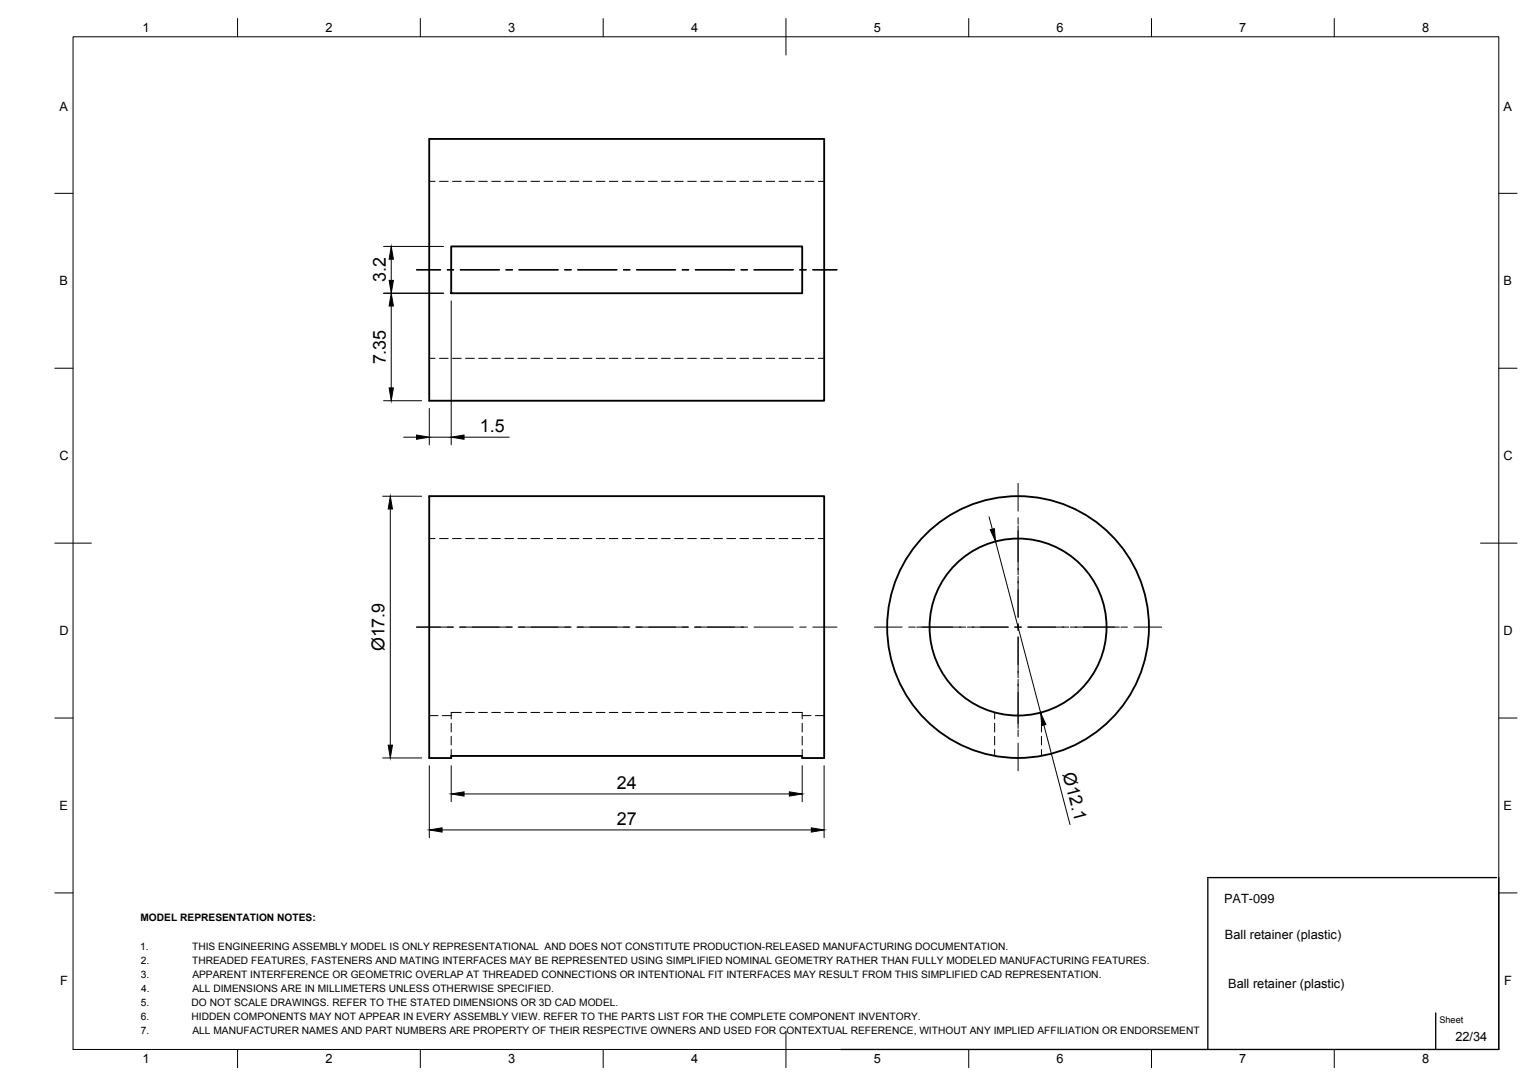
ISO-10303-21;
HEADER;
/* Generated by software containing ST-Developer
 * from STEP Tools, Inc. (www.steptools.com) 
 */

FILE_DESCRIPTION(
/* description */ ('PAT-099'),
/* implementation_level */ '2;1');

FILE_NAME(
/* name */ 'Ball retainer (plastic).step',
/* time_stamp */ '2026-10-29T17:25:42-07:00',
/* author */ (''),
/* organization */ (''),
/* preprocessor_version */ 'ST-DEVELOPER v20.2',
/* originating_system */ 'Autodesk Translation Framework v15.17.0.0',
/* authorisation */ '');

FILE_SCHEMA (('AUTOMOTIVE_DESIGN { 1 0 10303 214 3 1 1 }'));
ENDSEC;

DATA;
#10=MECHANICAL_DESIGN_GEOMETRIC_PRESENTATION_REPRESENTATION('',(#345),#11035);
#295=SHAPE_REPRESENTATION_RELATIONSHIP('SRR','None',#11164,#320);
#320=ADVANCED_BREP_SHAPE_REPRESENTATION('',(#378),#11014);
#345=STYLED_ITEM('',(#11379),#378);
#378=MANIFOLD_SOLID_BREP('Body1',#4713);
#485=FACE_BOUND('',#1151,.T.);
#486=FACE_BOUND('',#1153,.T.);
#487=FACE_BOUND('',#1155,.T.);
#488=FACE_BOUND('',#1157,.T.);
#573=PLANE('',#5293);
#574=PLANE('',#5296);
#575=PLANE('',#5297);
#576=PLANE('',#5300);
#577=PLANE('',#5301);
#578=PLANE('',#5306);
#781=FACE_OUTER_BOUND('',#1146,.T.);
#782=FACE_OUTER_BOUND('',#1147,.T.);
#783=FACE_OUTER_BOUND('',#1148,.T.);
#784=FACE_OUTER_BOUND('',#1149,.T.);
#785=FACE_OUTER_BOUND('',#1150,.T.);
#786=FACE_OUTER_BOUND('',#1152,.T.);
#787=FACE_OUTER_BOUND('',#1154,.T.);
#788=FACE_OUTER_BOUND('',#1156,.T.);
#1146=EDGE_LOOP('',(#3683,#3684,#3685,#3686));
#1147=EDGE_LOOP('',(#3687,#3688,#3689,#3690));
#1148=EDGE_LOOP('',(#3691,#3692,#3693,#3694));
#1149=EDGE_LOOP('',(#3695,#3696,#3697,#3698));
#1150=EDGE_LOOP('',(#3699));
#1151=EDGE_LOOP('',(#3700));
#1152=EDGE_LOOP('',(#3701,#3702,#3703,#3704));
#1153=EDGE_LOOP('',(#3705,#3706,#3707,#3708));
#1154=EDGE_LOOP('',(#3709));
#1155=EDGE_LOOP('',(#3710));
#1156=EDGE_LOOP('',(#3711,#3712,#3713,#3714));
#1157=EDGE_LOOP('',(#3715,#3716,#3717,#3718));
#1452=LINE('',#9819,#1704);
#1453=LINE('',#9822,#1705);
#1454=LINE('',#9825,#1706);
#1455=LINE('',#9827,#1707);
#1456=LINE('',#9828,#1708);
#1457=LINE('',#9834,#1709);
#1458=LINE('',#9836,#1710);
#1459=LINE('',#9837,#1711);
#1460=LINE('',#9846,#1712);
#1461=LINE('',#9851,#1713);
#1704=VECTOR('',#6335,1.);
#1705=VECTOR('',#6338,1.);
#1706=VECTOR('',#6341,1.);
#1707=VECTOR('',#6342,1.);
#1708=VECTOR('',#6343,1.);
#1709=VECTOR('',#6350,1.);
#1710=VECTOR('',#6353,1.);
#1711=VECTOR('',#6354,1.);
#1712=VECTOR('',#6365,0.895);
#1713=VECTOR('',#6372,0.605);
#1991=CIRCLE('',#5294,0.895);
#1992=CIRCLE('',#5295,0.605);
#1993=CIRCLE('',#5298,0.895);
#1994=CIRCLE('',#5299,0.605);
#1995=CIRCLE('',#5302,0.895);
#1996=CIRCLE('',#5303,0.605);
#1997=CIRCLE('',#5305,0.895);
#1998=CIRCLE('',#5307,0.605);
#2326=VERTEX_POINT('',#9815);
#2327=VERTEX_POINT('',#9816);
#2328=VERTEX_POINT('',#9818);
#2329=VERTEX_POINT('',#9820);
#2330=VERTEX_POINT('',#9824);
#2331=VERTEX_POINT('',#9826);
#2332=VERTEX_POINT('',#9830);
#2333=VERTEX_POINT('',#9832);
#2334=VERTEX_POINT('',#9839);
#2335=VERTEX_POINT('',#9841);
#2336=VERTEX_POINT('',#9844);
#2337=VERTEX_POINT('',#9848);
#2818=EDGE_CURVE('',#2326,#2327,#1991,.T.);
#2819=EDGE_CURVE('',#2328,#2326,#1452,.T.);
#2820=EDGE_CURVE('',#2329,#2328,#1992,.T.);
#2821=EDGE_CURVE('',#2327,#2329,#1453,.T.);
#2822=EDGE_CURVE('',#2327,#2330,#1454,.T.);
#2823=EDGE_CURVE('',#2331,#2329,#1455,.T.);
#2824=EDGE_CURVE('',#2331,#2330,#1456,.T.);
#2825=EDGE_CURVE('',#2330,#2332,#1993,.T.);
#2826=EDGE_CURVE('',#2333,#2331,#1994,.T.);
#2827=EDGE_CURVE('',#2332,#2333,#1457,.T.);
#2828=EDGE_CURVE('',#2332,#2326,#1458,.T.);
#2829=EDGE_CURVE('',#2328,#2333,#1459,.T.);
#2830=EDGE_CURVE('',#2334,#2334,#1995,.T.);
#2831=EDGE_CURVE('',#2335,#2335,#1996,.T.);
#2832=EDGE_CURVE('',#2336,#2336,#1997,.T.);
#2833=EDGE_CURVE('',#2336,#2334,#1460,.T.);
#2834=EDGE_CURVE('',#2337,#2337,#1998,.T.);
#2835=EDGE_CURVE('',#2337,#2335,#1461,.T.);
#3683=ORIENTED_EDGE('',*,*,#2818,.F.);
#3684=ORIENTED_EDGE('',*,*,#2819,.F.);
#3685=ORIENTED_EDGE('',*,*,#2820,.F.);
#3686=ORIENTED_EDGE('',*,*,#2821,.F.);
#3687=ORIENTED_EDGE('',*,*,#2822,.F.);
#3688=ORIENTED_EDGE('',*,*,#2821,.T.);
#3689=ORIENTED_EDGE('',*,*,#2823,.F.);
#3690=ORIENTED_EDGE('',*,*,#2824,.T.);
#3691=ORIENTED_EDGE('',*,*,#2825,.F.);
#3692=ORIENTED_EDGE('',*,*,#2824,.F.);
#3693=ORIENTED_EDGE('',*,*,#2826,.F.);
#3694=ORIENTED_EDGE('',*,*,#2827,.F.);
#3695=ORIENTED_EDGE('',*,*,#2828,.F.);
#3696=ORIENTED_EDGE('',*,*,#2827,.T.);
#3697=ORIENTED_EDGE('',*,*,#2829,.F.);
#3698=ORIENTED_EDGE('',*,*,#2819,.T.);
#3699=ORIENTED_EDGE('',*,*,#2830,.F.);
#3700=ORIENTED_EDGE('',*,*,#2831,.T.);
#3701=ORIENTED_EDGE('',*,*,#2832,.F.);
#3702=ORIENTED_EDGE('',*,*,#2833,.T.);
#3703=ORIENTED_EDGE('',*,*,#2830,.T.);
#3704=ORIENTED_EDGE('',*,*,#2833,.F.);
#3705=ORIENTED_EDGE('',*,*,#2825,.T.);
#3706=ORIENTED_EDGE('',*,*,#2828,.T.);
#3707=ORIENTED_EDGE('',*,*,#2818,.T.);
#3708=ORIENTED_EDGE('',*,*,#2822,.T.);
#3709=ORIENTED_EDGE('',*,*,#2832,.T.);
#3710=ORIENTED_EDGE('',*,*,#2834,.F.);
#3711=ORIENTED_EDGE('',*,*,#2834,.T.);
#3712=ORIENTED_EDGE('',*,*,#2835,.T.);
#3713=ORIENTED_EDGE('',*,*,#2831,.F.);
#3714=ORIENTED_EDGE('',*,*,#2835,.F.);
#3715=ORIENTED_EDGE('',*,*,#2826,.T.);
#3716=ORIENTED_EDGE('',*,*,#2823,.T.);
#3717=ORIENTED_EDGE('',*,*,#2820,.T.);
#3718=ORIENTED_EDGE('',*,*,#2829,.T.);
#4380=CYLINDRICAL_SURFACE('',#5304,0.895);
#4381=CYLINDRICAL_SURFACE('',#5308,0.605);
#4546=ADVANCED_FACE('',(#781),#573,.F.);
#4547=ADVANCED_FACE('',(#782),#574,.F.);
#4548=ADVANCED_FACE('',(#783),#575,.F.);
#4549=ADVANCED_FACE('',(#784),#576,.F.);
#4550=ADVANCED_FACE('',(#785,#485),#577,.T.);
#4551=ADVANCED_FACE('',(#786,#486),#4380,.T.);
#4552=ADVANCED_FACE('',(#787,#487),#578,.T.);
#4553=ADVANCED_FACE('',(#788,#488),#4381,.F.);
#4713=CLOSED_SHELL('',(#4546,#4547,#4548,#4549,#4550,#4551,#4552,#4553));
#5292=AXIS2_PLACEMENT_3D('',#9813,#6329,#6330);
#5293=AXIS2_PLACEMENT_3D('',#9814,#6331,#6332);
#5294=AXIS2_PLACEMENT_3D('',#9817,#6333,#6334);
#5295=AXIS2_PLACEMENT_3D('',#9821,#6336,#6337);
#5296=AXIS2_PLACEMENT_3D('',#9823,#6339,#6340);
#5297=AXIS2_PLACEMENT_3D('',#9829,#6344,#6345);
#5298=AXIS2_PLACEMENT_3D('',#9831,#6346,#6347);
#5299=AXIS2_PLACEMENT_3D('',#9833,#6348,#6349);
#5300=AXIS2_PLACEMENT_3D('',#9835,#6351,#6352);
#5301=AXIS2_PLACEMENT_3D('',#9838,#6355,#6356);
#5302=AXIS2_PLACEMENT_3D('',#9840,#6357,#6358);
#5303=AXIS2_PLACEMENT_3D('',#9842,#6359,#6360);
#5304=AXIS2_PLACEMENT_3D('',#9843,#6361,#6362);
#5305=AXIS2_PLACEMENT_3D('',#9845,#6363,#6364);
#5306=AXIS2_PLACEMENT_3D('',#9847,#6366,#6367);
#5307=AXIS2_PLACEMENT_3D('',#9849,#6368,#6369);
#5308=AXIS2_PLACEMENT_3D('',#9850,#6370,#6371);
#6329=DIRECTION('axis',(0.,0.,1.));
#6330=DIRECTION('refdir',(1.,0.,0.));
#6331=DIRECTION('center_axis',(0.,1.,0.));
#6332=DIRECTION('ref_axis',(0.,0.,1.));
#6333=DIRECTION('center_axis',(0.,1.,0.));
#6334=DIRECTION('ref_axis',(1.,0.,0.));
#6335=DIRECTION('',(1.,0.,0.));
#6336=DIRECTION('center_axis',(0.,-1.,0.));
#6337=DIRECTION('ref_axis',(1.,0.,0.));
#6338=DIRECTION('',(-1.,0.,0.));
#6339=DIRECTION('center_axis',(0.,0.,-1.));
#6340=DIRECTION('ref_axis',(-1.,0.,0.));
#6341=DIRECTION('',(0.,-1.,0.));
#6342=DIRECTION('',(0.,1.,0.));
#6343=DIRECTION('',(1.,0.,0.));
#6344=DIRECTION('center_axis',(0.,-1.,0.));
#6345=DIRECTION('ref_axis',(0.,0.,-1.));
#6346=DIRECTION('center_axis',(0.,-1.,0.));
#6347=DIRECTION('ref_axis',(1.,0.,0.));
#6348=DIRECTION('center_axis',(0.,1.,0.));
#6349=DIRECTION('ref_axis',(1.,0.,0.));
#6350=DIRECTION('',(-1.,0.,0.));
#6351=DIRECTION('center_axis',(0.,0.,1.));
#6352=DIRECTION('ref_axis',(1.,0.,0.));
#6353=DIRECTION('',(0.,1.,0.));
#6354=DIRECTION('',(0.,-1.,0.));
#6355=DIRECTION('center_axis',(0.,1.,0.));
#6356=DIRECTION('ref_axis',(0.,0.,1.));
#6357=DIRECTION('center_axis',(0.,-1.,0.));
#6358=DIRECTION('ref_axis',(1.,0.,0.));
#6359=DIRECTION('center_axis',(0.,-1.,0.));
#6360=DIRECTION('ref_axis',(1.,0.,0.));
#6361=DIRECTION('center_axis',(0.,-1.,0.));
#6362=DIRECTION('ref_axis',(1.,0.,0.));
#6363=DIRECTION('center_axis',(0.,-1.,0.));
#6364=DIRECTION('ref_axis',(1.,0.,0.));
#6365=DIRECTION('',(0.,1.,0.));
#6366=DIRECTION('center_axis',(0.,-1.,0.));
#6367=DIRECTION('ref_axis',(0.,0.,-1.));
#6368=DIRECTION('center_axis',(0.,-1.,0.));
#6369=DIRECTION('ref_axis',(1.,0.,0.));
#6370=DIRECTION('center_axis',(0.,-1.,0.));
#6371=DIRECTION('ref_axis',(1.,0.,0.));
#6372=DIRECTION('',(0.,1.,0.));
#9813=CARTESIAN_POINT('',(0.,0.,0.));
#9814=CARTESIAN_POINT('Origin',(0.75,1.2,0.));
#9815=CARTESIAN_POINT('',(0.880582193778639,1.2,0.16));
#9816=CARTESIAN_POINT('',(0.880582193778639,1.2,-0.16));
#9817=CARTESIAN_POINT('Origin',(0.,1.2,0.));
#9818=CARTESIAN_POINT('',(0.583459510163302,1.2,0.16));
#9819=CARTESIAN_POINT('',(0.57,1.2,0.16));
#9820=CARTESIAN_POINT('',(0.583459510163302,1.2,-0.16));
#9821=CARTESIAN_POINT('Origin',(0.,1.2,0.));
#9822=CARTESIAN_POINT('',(0.93,1.2,-0.16));
#9823=CARTESIAN_POINT('Origin',(0.93,0.,-0.16));
#9824=CARTESIAN_POINT('',(0.880582193778639,-1.2,-0.16));
#9825=CARTESIAN_POINT('',(0.880582193778639,0.,-0.16));
#9826=CARTESIAN_POINT('',(0.583459510163302,-1.2,-0.16));
#9827=CARTESIAN_POINT('',(0.583459510163302,0.,-0.16));
#9828=CARTESIAN_POINT('',(0.93,-1.2,-0.16));
#9829=CARTESIAN_POINT('Origin',(0.75,-1.2,0.));
#9830=CARTESIAN_POINT('',(0.880582193778639,-1.2,0.16));
#9831=CARTESIAN_POINT('Origin',(0.,-1.2,0.));
#9832=CARTESIAN_POINT('',(0.583459510163302,-1.2,0.16));
#9833=CARTESIAN_POINT('Origin',(0.,-1.2,0.));
#9834=CARTESIAN_POINT('',(0.57,-1.2,0.16));
#9835=CARTESIAN_POINT('Origin',(0.57,0.,0.16));
#9836=CARTESIAN_POINT('',(0.880582193778639,0.,0.16));
#9837=CARTESIAN_POINT('',(0.583459510163302,0.,0.16));
#9838=CARTESIAN_POINT('Origin',(0.895,1.35,0.));
#9839=CARTESIAN_POINT('',(-0.895,1.35,-1.09605888523688E-16));
#9840=CARTESIAN_POINT('Origin',(0.,1.35,0.));
#9841=CARTESIAN_POINT('',(-0.605,1.35,-7.40911313484149E-17));
#9842=CARTESIAN_POINT('Origin',(0.,1.35,0.));
#9843=CARTESIAN_POINT('Origin',(0.,0.,0.));
#9844=CARTESIAN_POINT('',(-0.895,-1.35,-1.09605888523688E-16));
#9845=CARTESIAN_POINT('Origin',(0.,-1.35,0.));
#9846=CARTESIAN_POINT('',(-0.895,0.,-1.09605888523688E-16));
#9847=CARTESIAN_POINT('Origin',(0.605,-1.35,0.));
#9848=CARTESIAN_POINT('',(-0.605,-1.35,-7.40911313484149E-17));
#9849=CARTESIAN_POINT('Origin',(0.,-1.35,0.));
#9850=CARTESIAN_POINT('Origin',(0.,0.,0.));
#9851=CARTESIAN_POINT('',(-0.605,0.,-7.40911313484149E-17));
#10981=UNCERTAINTY_MEASURE_WITH_UNIT(LENGTH_MEASURE(0.001),#11036,
'DISTANCE_ACCURACY_VALUE',
'Maximum model space distance between geometric entities at asserted c
onnectivities');
#11002=UNCERTAINTY_MEASURE_WITH_UNIT(LENGTH_MEASURE(0.001),#11036,
'DISTANCE_ACCURACY_VALUE',
'Maximum model space distance between geometric entities at asserted c
onnectivities');
#11014=(
GEOMETRIC_REPRESENTATION_CONTEXT(3)
GLOBAL_UNCERTAINTY_ASSIGNED_CONTEXT((#10981))
GLOBAL_UNIT_ASSIGNED_CONTEXT((#11036,#11038,#11039))
REPRESENTATION_CONTEXT('','3D')
);
#11035=(
GEOMETRIC_REPRESENTATION_CONTEXT(3)
GLOBAL_UNCERTAINTY_ASSIGNED_CONTEXT((#11002))
GLOBAL_UNIT_ASSIGNED_CONTEXT((#11036,#11038,#11039))
REPRESENTATION_CONTEXT('','3D')
);
#11036=(
LENGTH_UNIT()
NAMED_UNIT(*)
SI_UNIT(.CENTI.,.METRE.)
);
#11038=(
NAMED_UNIT(*)
PLANE_ANGLE_UNIT()
SI_UNIT($,.RADIAN.)
);
#11039=(
NAMED_UNIT(*)
SI_UNIT($,.STERADIAN.)
SOLID_ANGLE_UNIT()
);
#11051=SHAPE_DEFINITION_REPRESENTATION(#11083,#11164);
#11083=PRODUCT_DEFINITION_SHAPE('',$,#11197);
#11164=SHAPE_REPRESENTATION('',(#5292),#11014);
#11185=PRODUCT_DEFINITION_CONTEXT('part definition',#11283,'design');
#11197=PRODUCT_DEFINITION('Ball retainer (plastic)',
'Ball retainer (plastic)',#11229,#11185);
#11229=PRODUCT_DEFINITION_FORMATION('',$,#11296);
#11283=APPLICATION_CONTEXT(
'Core Data for Automotive Mechanical Design Process');
#11284=PRODUCT_CONTEXT('part definition',#11283,'mechanical');
#11296=PRODUCT('Ball retainer (plastic)','Ball retainer (plastic)',
'Ball retainer (plastic)',(#11284));
#11373=COLOUR_RGB('Sky Blue',0.24,0.69,0.87);
#11374=FILL_AREA_STYLE_COLOUR('',#11373);
#11375=FILL_AREA_STYLE('',(#11374));
#11376=SURFACE_STYLE_FILL_AREA(#11375);
#11377=SURFACE_SIDE_STYLE('',(#11376));
#11378=SURFACE_STYLE_USAGE(.BOTH.,#11377);
#11379=PRESENTATION_STYLE_ASSIGNMENT((#11378));
ENDSEC;
END-ISO-10303-21;
